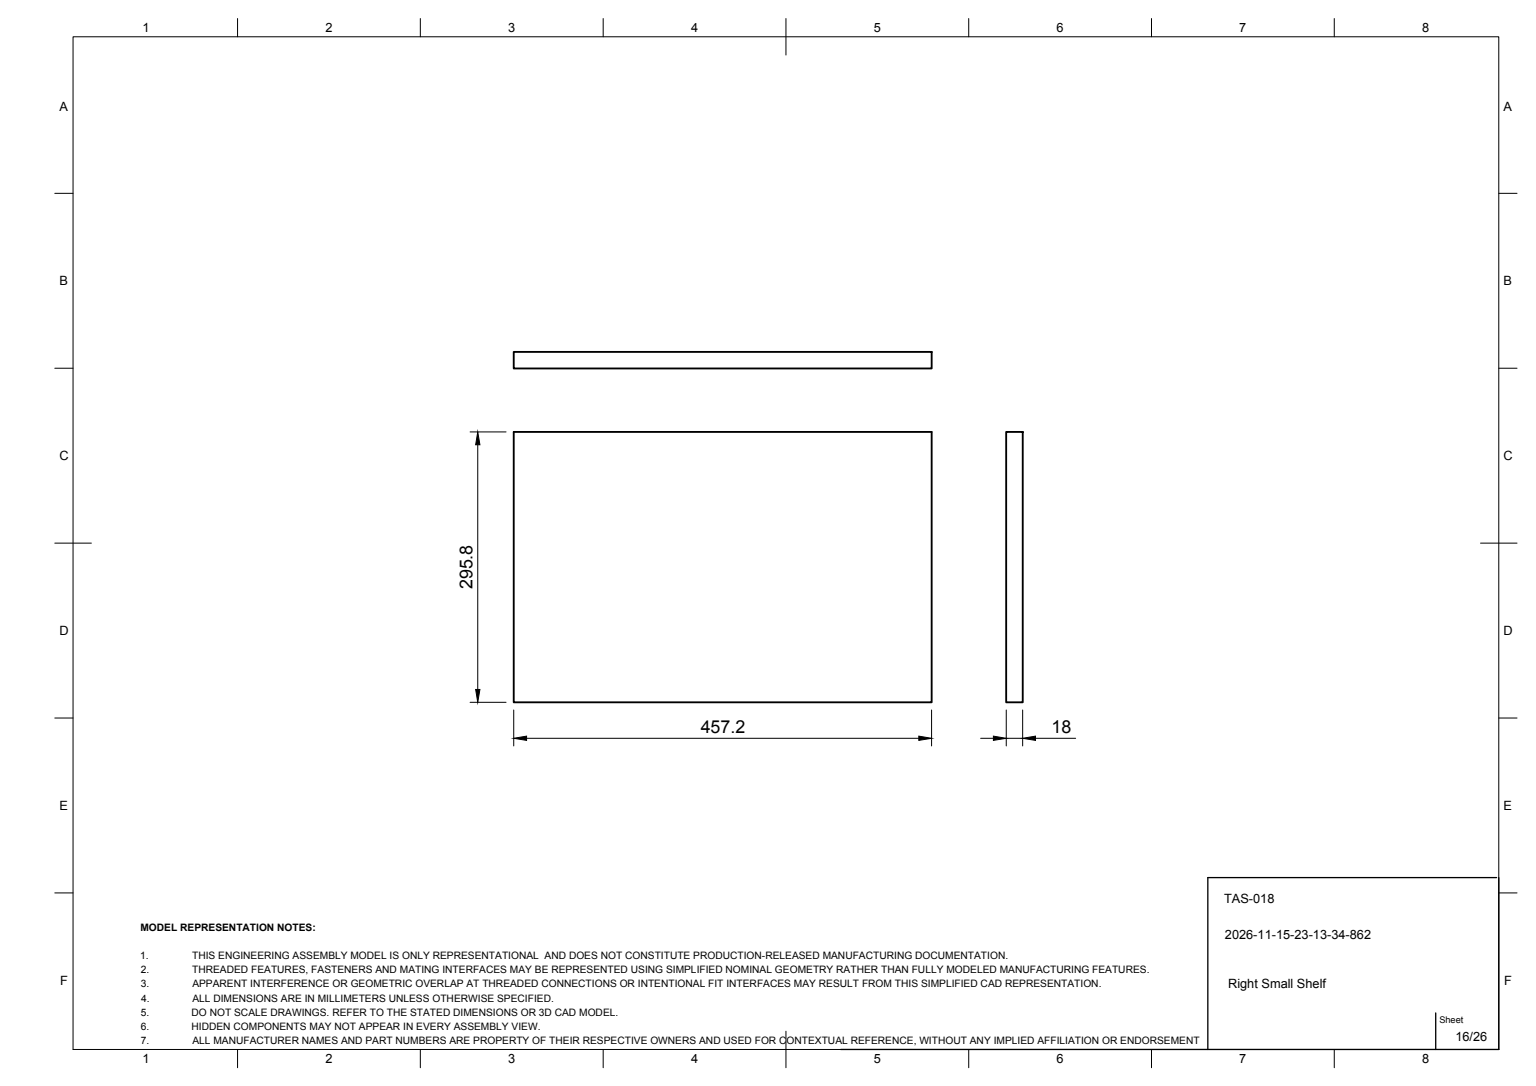
ISO-10303-21;
HEADER;
/* Generated by software containing ST-Developer
 * from STEP Tools, Inc. (www.steptools.com) 
 */

FILE_DESCRIPTION(
/* description */ (''),
/* implementation_level */ '2;1');

FILE_NAME(
/* name */ 'Right Small Shelf.step',
/* time_stamp */ '2026-11-15T15:17:57-08:00',
/* author */ (''),
/* organization */ (''),
/* preprocessor_version */ 'ST-DEVELOPER v20.2',
/* originating_system */ 'Autodesk Translation Framework v15.17.0.0',
/* authorisation */ '');

FILE_SCHEMA (('AUTOMOTIVE_DESIGN { 1 0 10303 214 3 1 1 }'));
ENDSEC;

DATA;
#10=MECHANICAL_DESIGN_GEOMETRIC_PRESENTATION_REPRESENTATION('',(#191),#3723);
#143=SHAPE_REPRESENTATION_RELATIONSHIP('SRR','None',#3824,#167);
#167=ADVANCED_BREP_SHAPE_REPRESENTATION('',(#215),#3713);
#191=STYLED_ITEM('',(#3944),#215);
#215=MANIFOLD_SOLID_BREP('Body1',#2039);
#303=FACE_OUTER_BOUND('',#429,.T.);
#304=FACE_OUTER_BOUND('',#430,.T.);
#305=FACE_OUTER_BOUND('',#431,.T.);
#306=FACE_OUTER_BOUND('',#432,.T.);
#307=FACE_OUTER_BOUND('',#433,.T.);
#308=FACE_OUTER_BOUND('',#434,.T.);
#429=EDGE_LOOP('',(#1611,#1612,#1613,#1614));
#430=EDGE_LOOP('',(#1615,#1616,#1617,#1618));
#431=EDGE_LOOP('',(#1619,#1620,#1621,#1622));
#432=EDGE_LOOP('',(#1623,#1624,#1625,#1626));
#433=EDGE_LOOP('',(#1627,#1628,#1629,#1630));
#434=EDGE_LOOP('',(#1631,#1632,#1633,#1634));
#623=LINE('',#3452,#845);
#624=LINE('',#3454,#846);
#625=LINE('',#3456,#847);
#626=LINE('',#3457,#848);
#627=LINE('',#3460,#849);
#628=LINE('',#3462,#850);
#629=LINE('',#3463,#851);
#630=LINE('',#3466,#852);
#631=LINE('',#3468,#853);
#632=LINE('',#3469,#854);
#633=LINE('',#3471,#855);
#634=LINE('',#3472,#856);
#845=VECTOR('',#2851,0.708661417322833);
#846=VECTOR('',#2852,18.);
#847=VECTOR('',#2853,0.708661417322833);
#848=VECTOR('',#2854,18.);
#849=VECTOR('',#2857,11.6456692913386);
#850=VECTOR('',#2858,11.6456692913386);
#851=VECTOR('',#2859,18.);
#852=VECTOR('',#2862,0.708661417322845);
#853=VECTOR('',#2863,0.708661417322845);
#854=VECTOR('',#2864,18.);
#855=VECTOR('',#2867,11.6456692913386);
#856=VECTOR('',#2868,11.6456692913386);
#1021=VERTEX_POINT('',#3450);
#1022=VERTEX_POINT('',#3451);
#1023=VERTEX_POINT('',#3453);
#1024=VERTEX_POINT('',#3455);
#1025=VERTEX_POINT('',#3459);
#1026=VERTEX_POINT('',#3461);
#1027=VERTEX_POINT('',#3465);
#1028=VERTEX_POINT('',#3467);
#1227=EDGE_CURVE('',#1021,#1022,#623,.T.);
#1228=EDGE_CURVE('',#1021,#1023,#624,.T.);
#1229=EDGE_CURVE('',#1023,#1024,#625,.T.);
#1230=EDGE_CURVE('',#1022,#1024,#626,.T.);
#1231=EDGE_CURVE('',#1022,#1025,#627,.T.);
#1232=EDGE_CURVE('',#1024,#1026,#628,.T.);
#1233=EDGE_CURVE('',#1025,#1026,#629,.T.);
#1234=EDGE_CURVE('',#1025,#1027,#630,.T.);
#1235=EDGE_CURVE('',#1026,#1028,#631,.T.);
#1236=EDGE_CURVE('',#1027,#1028,#632,.T.);
#1237=EDGE_CURVE('',#1027,#1021,#633,.T.);
#1238=EDGE_CURVE('',#1028,#1023,#634,.T.);
#1611=ORIENTED_EDGE('',*,*,#1227,.F.);
#1612=ORIENTED_EDGE('',*,*,#1228,.T.);
#1613=ORIENTED_EDGE('',*,*,#1229,.T.);
#1614=ORIENTED_EDGE('',*,*,#1230,.F.);
#1615=ORIENTED_EDGE('',*,*,#1231,.F.);
#1616=ORIENTED_EDGE('',*,*,#1230,.T.);
#1617=ORIENTED_EDGE('',*,*,#1232,.T.);
#1618=ORIENTED_EDGE('',*,*,#1233,.F.);
#1619=ORIENTED_EDGE('',*,*,#1234,.F.);
#1620=ORIENTED_EDGE('',*,*,#1233,.T.);
#1621=ORIENTED_EDGE('',*,*,#1235,.T.);
#1622=ORIENTED_EDGE('',*,*,#1236,.F.);
#1623=ORIENTED_EDGE('',*,*,#1237,.F.);
#1624=ORIENTED_EDGE('',*,*,#1236,.T.);
#1625=ORIENTED_EDGE('',*,*,#1238,.T.);
#1626=ORIENTED_EDGE('',*,*,#1228,.F.);
#1627=ORIENTED_EDGE('',*,*,#1229,.F.);
#1628=ORIENTED_EDGE('',*,*,#1238,.F.);
#1629=ORIENTED_EDGE('',*,*,#1235,.F.);
#1630=ORIENTED_EDGE('',*,*,#1232,.F.);
#1631=ORIENTED_EDGE('',*,*,#1237,.T.);
#1632=ORIENTED_EDGE('',*,*,#1227,.T.);
#1633=ORIENTED_EDGE('',*,*,#1231,.T.);
#1634=ORIENTED_EDGE('',*,*,#1234,.T.);
#1855=PLANE('',#2414);
#1856=PLANE('',#2415);
#1857=PLANE('',#2416);
#1858=PLANE('',#2417);
#1859=PLANE('',#2418);
#1860=PLANE('',#2419);
#1977=ADVANCED_FACE('',(#303),#1855,.F.);
#1978=ADVANCED_FACE('',(#304),#1856,.F.);
#1979=ADVANCED_FACE('',(#305),#1857,.F.);
#1980=ADVANCED_FACE('',(#306),#1858,.F.);
#1981=ADVANCED_FACE('',(#307),#1859,.F.);
#1982=ADVANCED_FACE('',(#308),#1860,.T.);
#2039=CLOSED_SHELL('',(#1977,#1978,#1979,#1980,#1981,#1982));
#2413=AXIS2_PLACEMENT_3D('',#3448,#2847,#2848);
#2414=AXIS2_PLACEMENT_3D('',#3449,#2849,#2850);
#2415=AXIS2_PLACEMENT_3D('',#3458,#2855,#2856);
#2416=AXIS2_PLACEMENT_3D('',#3464,#2860,#2861);
#2417=AXIS2_PLACEMENT_3D('',#3470,#2865,#2866);
#2418=AXIS2_PLACEMENT_3D('',#3473,#2869,#2870);
#2419=AXIS2_PLACEMENT_3D('',#3474,#2871,#2872);
#2847=DIRECTION('axis',(0.,0.,1.));
#2848=DIRECTION('refdir',(1.,0.,0.));
#2849=DIRECTION('center_axis',(-1.,0.,0.));
#2850=DIRECTION('ref_axis',(0.,0.,1.));
#2851=DIRECTION('',(0.,1.,0.));
#2852=DIRECTION('',(0.,0.,-1.));
#2853=DIRECTION('',(0.,1.,0.));
#2854=DIRECTION('',(0.,0.,-1.));
#2855=DIRECTION('center_axis',(-7.50657893593751E-16,-1.,0.));
#2856=DIRECTION('ref_axis',(0.,0.,-1.));
#2857=DIRECTION('',(-1.,9.60842103800001E-16,0.));
#2858=DIRECTION('',(-1.,9.60842103800001E-16,0.));
#2859=DIRECTION('',(0.,0.,-1.));
#2860=DIRECTION('center_axis',(1.,0.,0.));
#2861=DIRECTION('ref_axis',(0.,0.,-1.));
#2862=DIRECTION('',(0.,-1.,0.));
#2863=DIRECTION('',(0.,-1.,0.));
#2864=DIRECTION('',(0.,0.,-1.));
#2865=DIRECTION('center_axis',(0.,1.,0.));
#2866=DIRECTION('ref_axis',(0.,0.,1.));
#2867=DIRECTION('',(1.,0.,0.));
#2868=DIRECTION('',(1.,0.,0.));
#2869=DIRECTION('center_axis',(0.,0.,1.));
#2870=DIRECTION('ref_axis',(1.,0.,0.));
#2871=DIRECTION('center_axis',(0.,0.,1.));
#2872=DIRECTION('ref_axis',(1.,0.,0.));
#3448=CARTESIAN_POINT('',(0.,0.,0.));
#3449=CARTESIAN_POINT('Origin',(35.2913385826772,48.6771653543307,30.375872491424));
#3450=CARTESIAN_POINT('',(35.2913385826772,47.9685039370079,18.7086614173228));
#3451=CARTESIAN_POINT('',(35.2913385826772,48.6771653543307,18.7086614173228));
#3452=CARTESIAN_POINT('',(35.2913385826772,47.9685039370079,18.7086614173228));
#3453=CARTESIAN_POINT('',(35.2913385826772,47.9685039370079,0.708661417322834));
#3454=CARTESIAN_POINT('',(35.2913385826772,47.9685039370079,18.7086614173228));
#3455=CARTESIAN_POINT('',(35.2913385826772,48.6771653543307,0.708661417322834));
#3456=CARTESIAN_POINT('',(35.2913385826772,47.9685039370079,0.708661417322834));
#3457=CARTESIAN_POINT('',(35.2913385826772,48.6771653543307,18.7086614173228));
#3458=CARTESIAN_POINT('Origin',(23.6456692913386,48.6771653543307,30.375872491424));
#3459=CARTESIAN_POINT('',(23.6456692913386,48.6771653543307,18.7086614173228));
#3460=CARTESIAN_POINT('',(35.2913385826772,48.6771653543307,18.7086614173228));
#3461=CARTESIAN_POINT('',(23.6456692913386,48.6771653543307,0.708661417322834));
#3462=CARTESIAN_POINT('',(35.2913385826771,48.6771653543307,0.708661417322834));
#3463=CARTESIAN_POINT('',(23.6456692913386,48.6771653543307,18.7086614173228));
#3464=CARTESIAN_POINT('Origin',(23.6456692913386,48.6771653543307,30.375872491424));
#3465=CARTESIAN_POINT('',(23.6456692913386,47.9685039370079,18.7086614173228));
#3466=CARTESIAN_POINT('',(23.6456692913386,48.6771653543307,18.7086614173228));
#3467=CARTESIAN_POINT('',(23.6456692913386,47.9685039370079,0.708661417322834));
#3468=CARTESIAN_POINT('',(23.6456692913386,48.6771653543307,0.708661417322834));
#3469=CARTESIAN_POINT('',(23.6456692913386,47.9685039370079,18.7086614173228));
#3470=CARTESIAN_POINT('Origin',(23.6456692913386,47.9685039370079,30.375872491424));
#3471=CARTESIAN_POINT('',(23.6456692913386,47.9685039370079,18.7086614173228));
#3472=CARTESIAN_POINT('',(23.6456692913386,47.9685039370079,0.708661417322834));
#3473=CARTESIAN_POINT('Origin',(0.,0.,0.708661417322834));
#3474=CARTESIAN_POINT('Origin',(0.,0.,18.7086614173228));
#3686=UNCERTAINTY_MEASURE_WITH_UNIT(LENGTH_MEASURE(0.000393700787401575),
#3725,'DISTANCE_ACCURACY_VALUE',
'Maximum model space distance between geometric entities at asserted c
onnectivities');
#3696=UNCERTAINTY_MEASURE_WITH_UNIT(LENGTH_MEASURE(0.000393700787401575),
#3725,'DISTANCE_ACCURACY_VALUE',
'Maximum model space distance between geometric entities at asserted c
onnectivities');
#3713=(
GEOMETRIC_REPRESENTATION_CONTEXT(3)
GLOBAL_UNCERTAINTY_ASSIGNED_CONTEXT((#3686))
GLOBAL_UNIT_ASSIGNED_CONTEXT((#3725,#3729,#3730))
REPRESENTATION_CONTEXT('','3D')
);
#3723=(
GEOMETRIC_REPRESENTATION_CONTEXT(3)
GLOBAL_UNCERTAINTY_ASSIGNED_CONTEXT((#3696))
GLOBAL_UNIT_ASSIGNED_CONTEXT((#3725,#3729,#3730))
REPRESENTATION_CONTEXT('','3D')
);
#3724=DIMENSIONAL_EXPONENTS(1.,0.,0.,0.,0.,0.,0.);
#3725=(
CONVERSION_BASED_UNIT('inch',#3728)
LENGTH_UNIT()
NAMED_UNIT(#3724)
);
#3726=(
LENGTH_UNIT()
NAMED_UNIT(*)
SI_UNIT(.MILLI.,.METRE.)
);
#3728=LENGTH_MEASURE_WITH_UNIT(LENGTH_MEASURE(25.4),#3726);
#3729=(
NAMED_UNIT(*)
PLANE_ANGLE_UNIT()
SI_UNIT($,.RADIAN.)
);
#3730=(
NAMED_UNIT(*)
SI_UNIT($,.STERADIAN.)
SOLID_ANGLE_UNIT()
);
#3747=SHAPE_DEFINITION_REPRESENTATION(#3774,#3824);
#3774=PRODUCT_DEFINITION_SHAPE('',$,#3851);
#3824=SHAPE_REPRESENTATION('',(#2413),#3713);
#3834=PRODUCT_DEFINITION_CONTEXT('part definition',#3914,'design');
#3851=PRODUCT_DEFINITION('2026-11-15-23-13-34-862','Right Small Shelf',
#3877,#3834);
#3877=PRODUCT_DEFINITION_FORMATION('',$,#3932);
#3914=APPLICATION_CONTEXT(
'Core Data for Automotive Mechanical Design Process');
#3915=PRODUCT_CONTEXT('part definition',#3914,'mechanical');
#3932=PRODUCT('2026-11-15-23-13-34-862','Right Small Shelf',$,(#3915));
#3944=PRESENTATION_STYLE_ASSIGNMENT((#3952));
#3952=SURFACE_STYLE_USAGE(.BOTH.,#3960);
#3960=SURFACE_SIDE_STYLE('',(#3968));
#3968=SURFACE_STYLE_FILL_AREA(#3976);
#3976=FILL_AREA_STYLE('Light Gray',(#3984));
#3984=FILL_AREA_STYLE_COLOUR('Light Gray',#3992);
#3992=COLOUR_RGB('Light Gray',0.827450980392157,0.827450980392157,0.827450980392157);
ENDSEC;
END-ISO-10303-21;
